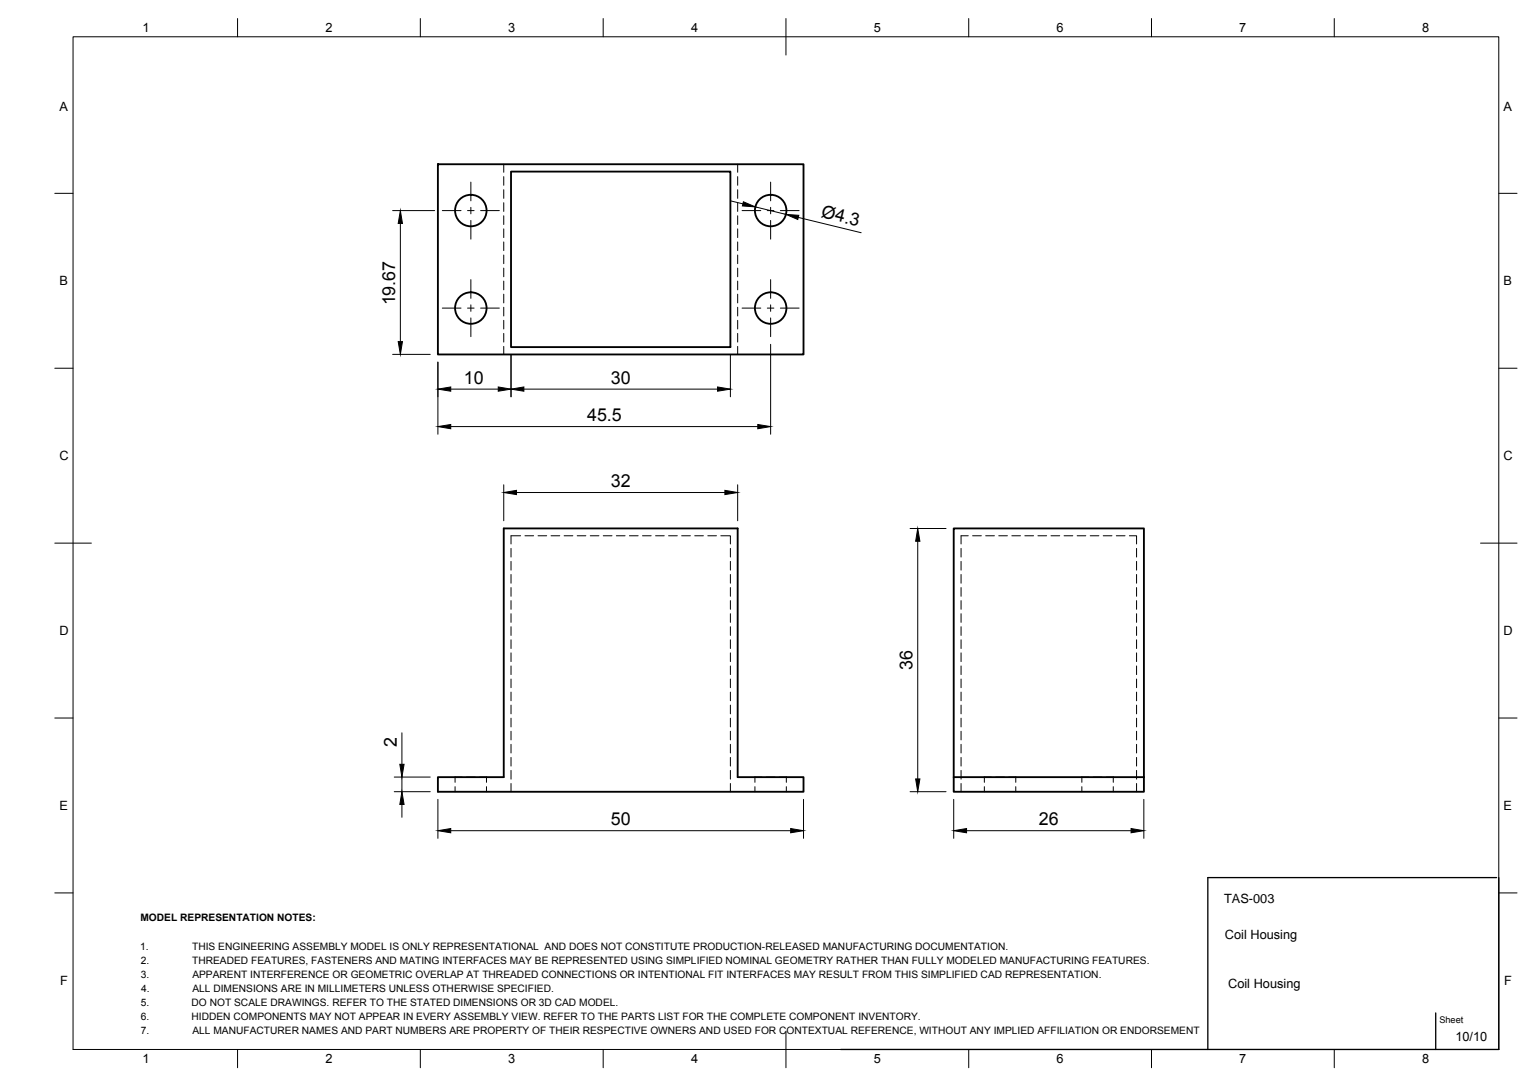
ISO-10303-21;
HEADER;
/* Generated by software containing ST-Developer
 * from STEP Tools, Inc. (www.steptools.com) 
 */

FILE_DESCRIPTION(
/* description */ ('STEP AP214'),
/* implementation_level */ '2;1');

FILE_NAME(
/* name */ 'Coil Housing.step',
/* time_stamp */ '2026-11-04T19:43:37-08:00',
/* author */ (''),
/* organization */ (''),
/* preprocessor_version */ 'ST-DEVELOPER v20.2',
/* originating_system */ 'Autodesk Translation Framework v15.17.0.0',
/* authorisation */ '');

FILE_SCHEMA (('AUTOMOTIVE_DESIGN { 1 0 10303 214 3 1 1 }'));
ENDSEC;

DATA;
#10=MECHANICAL_DESIGN_GEOMETRIC_PRESENTATION_REPRESENTATION('',(#134),#7627);
#86=TOROIDAL_SURFACE('',#2777,2.2,0.2);
#87=TOROIDAL_SURFACE('',#2781,2.2,0.2);
#88=TOROIDAL_SURFACE('',#2785,2.2,0.2);
#89=TOROIDAL_SURFACE('',#2789,2.2,0.2);
#104=SHAPE_REPRESENTATION_RELATIONSHIP('SRR','None',#7672,#113);
#113=ADVANCED_BREP_SHAPE_REPRESENTATION('',(#155),#7625);
#134=STYLED_ITEM('',(#7719),#155);
#155=MANIFOLD_SOLID_BREP('Body1',#2432);
#179=FACE_BOUND('',#605,.T.);
#180=FACE_BOUND('',#606,.T.);
#181=FACE_BOUND('',#607,.T.);
#182=FACE_BOUND('',#608,.T.);
#183=FACE_BOUND('',#609,.T.);
#184=FACE_BOUND('',#620,.T.);
#185=FACE_BOUND('',#621,.T.);
#186=FACE_BOUND('',#624,.T.);
#187=FACE_BOUND('',#625,.T.);
#222=PLANE('',#2801);
#223=PLANE('',#2802);
#224=PLANE('',#2803);
#225=PLANE('',#2804);
#226=PLANE('',#2805);
#227=PLANE('',#2806);
#228=PLANE('',#2807);
#229=PLANE('',#2808);
#230=PLANE('',#2809);
#231=PLANE('',#2810);
#232=PLANE('',#2811);
#233=PLANE('',#2812);
#234=PLANE('',#2813);
#235=PLANE('',#2814);
#236=PLANE('',#2815);
#302=CYLINDRICAL_SURFACE('',#2793,2.15);
#303=CYLINDRICAL_SURFACE('',#2795,2.15);
#304=CYLINDRICAL_SURFACE('',#2797,2.15);
#305=CYLINDRICAL_SURFACE('',#2799,2.15);
#418=FACE_OUTER_BOUND('',#594,.T.);
#419=FACE_OUTER_BOUND('',#595,.T.);
#420=FACE_OUTER_BOUND('',#596,.T.);
#421=FACE_OUTER_BOUND('',#597,.T.);
#422=FACE_OUTER_BOUND('',#598,.T.);
#423=FACE_OUTER_BOUND('',#599,.T.);
#424=FACE_OUTER_BOUND('',#600,.T.);
#425=FACE_OUTER_BOUND('',#601,.T.);
#426=FACE_OUTER_BOUND('',#602,.T.);
#427=FACE_OUTER_BOUND('',#603,.T.);
#428=FACE_OUTER_BOUND('',#604,.T.);
#429=FACE_OUTER_BOUND('',#610,.T.);
#430=FACE_OUTER_BOUND('',#611,.T.);
#431=FACE_OUTER_BOUND('',#612,.T.);
#432=FACE_OUTER_BOUND('',#613,.T.);
#433=FACE_OUTER_BOUND('',#614,.T.);
#434=FACE_OUTER_BOUND('',#615,.T.);
#435=FACE_OUTER_BOUND('',#616,.T.);
#436=FACE_OUTER_BOUND('',#617,.T.);
#437=FACE_OUTER_BOUND('',#618,.T.);
#438=FACE_OUTER_BOUND('',#619,.T.);
#439=FACE_OUTER_BOUND('',#622,.T.);
#440=FACE_OUTER_BOUND('',#623,.T.);
#594=EDGE_LOOP('',(#2057,#2058,#2059,#2060));
#595=EDGE_LOOP('',(#2061,#2062,#2063,#2064));
#596=EDGE_LOOP('',(#2065,#2066,#2067,#2068));
#597=EDGE_LOOP('',(#2069,#2070,#2071,#2072));
#598=EDGE_LOOP('',(#2073,#2074,#2075,#2076));
#599=EDGE_LOOP('',(#2077,#2078,#2079,#2080));
#600=EDGE_LOOP('',(#2081,#2082,#2083,#2084));
#601=EDGE_LOOP('',(#2085,#2086,#2087,#2088));
#602=EDGE_LOOP('',(#2089,#2090,#2091,#2092));
#603=EDGE_LOOP('',(#2093,#2094,#2095,#2096));
#604=EDGE_LOOP('',(#2097,#2098,#2099,#2100));
#605=EDGE_LOOP('',(#2101,#2102,#2103,#2104));
#606=EDGE_LOOP('',(#2105));
#607=EDGE_LOOP('',(#2106));
#608=EDGE_LOOP('',(#2107));
#609=EDGE_LOOP('',(#2108));
#610=EDGE_LOOP('',(#2109,#2110,#2111,#2112,#2113,#2114,#2115,#2116));
#611=EDGE_LOOP('',(#2117,#2118,#2119,#2120,#2121,#2122,#2123,#2124));
#612=EDGE_LOOP('',(#2125,#2126,#2127,#2128));
#613=EDGE_LOOP('',(#2129,#2130,#2131,#2132));
#614=EDGE_LOOP('',(#2133,#2134,#2135,#2136));
#615=EDGE_LOOP('',(#2137,#2138,#2139,#2140));
#616=EDGE_LOOP('',(#2141,#2142,#2143,#2144));
#617=EDGE_LOOP('',(#2145,#2146,#2147,#2148));
#618=EDGE_LOOP('',(#2149,#2150,#2151,#2152));
#619=EDGE_LOOP('',(#2153,#2154,#2155,#2156));
#620=EDGE_LOOP('',(#2157));
#621=EDGE_LOOP('',(#2158));
#622=EDGE_LOOP('',(#2159,#2160,#2161,#2162));
#623=EDGE_LOOP('',(#2163,#2164,#2165,#2166));
#624=EDGE_LOOP('',(#2167));
#625=EDGE_LOOP('',(#2168));
#773=CIRCLE('',#2778,2.15);
#774=CIRCLE('',#2779,0.2);
#775=CIRCLE('',#2780,2.2);
#776=CIRCLE('',#2782,2.15);
#777=CIRCLE('',#2783,0.2);
#778=CIRCLE('',#2784,2.2);
#779=CIRCLE('',#2786,2.15);
#780=CIRCLE('',#2787,0.2);
#781=CIRCLE('',#2788,2.2);
#782=CIRCLE('',#2790,2.15);
#783=CIRCLE('',#2791,0.2);
#784=CIRCLE('',#2792,2.2);
#785=CIRCLE('',#2794,2.15);
#786=CIRCLE('',#2796,2.15);
#787=CIRCLE('',#2798,2.15);
#788=CIRCLE('',#2800,2.15);
#891=LINE('',#7416,#1047);
#892=LINE('',#7420,#1048);
#893=LINE('',#7424,#1049);
#894=LINE('',#7428,#1050);
#895=LINE('',#7432,#1051);
#896=LINE('',#7434,#1052);
#897=LINE('',#7436,#1053);
#898=LINE('',#7437,#1054);
#899=LINE('',#7441,#1055);
#900=LINE('',#7443,#1056);
#901=LINE('',#7445,#1057);
#902=LINE('',#7446,#1058);
#903=LINE('',#7450,#1059);
#904=LINE('',#7452,#1060);
#905=LINE('',#7454,#1061);
#906=LINE('',#7455,#1062);
#907=LINE('',#7458,#1063);
#908=LINE('',#7460,#1064);
#909=LINE('',#7462,#1065);
#910=LINE('',#7463,#1066);
#911=LINE('',#7466,#1067);
#912=LINE('',#7467,#1068);
#913=LINE('',#7468,#1069);
#914=LINE('',#7470,#1070);
#915=LINE('',#7471,#1071);
#916=LINE('',#7474,#1072);
#917=LINE('',#7475,#1073);
#918=LINE('',#7476,#1074);
#919=LINE('',#7478,#1075);
#920=LINE('',#7479,#1076);
#921=LINE('',#7482,#1077);
#922=LINE('',#7484,#1078);
#923=LINE('',#7485,#1079);
#924=LINE('',#7488,#1080);
#925=LINE('',#7489,#1081);
#926=LINE('',#7492,#1082);
#927=LINE('',#7493,#1083);
#928=LINE('',#7495,#1084);
#929=LINE('',#7499,#1085);
#930=LINE('',#7502,#1086);
#1047=VECTOR('',#3474,2.15);
#1048=VECTOR('',#3479,2.15);
#1049=VECTOR('',#3484,2.15);
#1050=VECTOR('',#3489,2.15);
#1051=VECTOR('',#3492,1000.);
#1052=VECTOR('',#3493,1000.);
#1053=VECTOR('',#3494,1000.);
#1054=VECTOR('',#3495,1000.);
#1055=VECTOR('',#3498,1000.);
#1056=VECTOR('',#3499,1000.);
#1057=VECTOR('',#3500,1000.);
#1058=VECTOR('',#3501,1000.);
#1059=VECTOR('',#3504,1000.);
#1060=VECTOR('',#3505,1000.);
#1061=VECTOR('',#3506,1000.);
#1062=VECTOR('',#3507,1000.);
#1063=VECTOR('',#3508,1000.);
#1064=VECTOR('',#3509,1000.);
#1065=VECTOR('',#3510,1000.);
#1066=VECTOR('',#3511,1000.);
#1067=VECTOR('',#3514,1000.);
#1068=VECTOR('',#3515,1000.);
#1069=VECTOR('',#3516,1000.);
#1070=VECTOR('',#3517,1000.);
#1071=VECTOR('',#3518,1000.);
#1072=VECTOR('',#3521,1000.);
#1073=VECTOR('',#3522,1000.);
#1074=VECTOR('',#3523,1000.);
#1075=VECTOR('',#3524,1000.);
#1076=VECTOR('',#3525,1000.);
#1077=VECTOR('',#3528,1000.);
#1078=VECTOR('',#3529,1000.);
#1079=VECTOR('',#3530,1000.);
#1080=VECTOR('',#3533,1000.);
#1081=VECTOR('',#3534,1000.);
#1082=VECTOR('',#3537,1000.);
#1083=VECTOR('',#3538,1000.);
#1084=VECTOR('',#3541,1000.);
#1085=VECTOR('',#3548,1000.);
#1086=VECTOR('',#3553,1000.);
#1243=VERTEX_POINT('',#7390);
#1244=VERTEX_POINT('',#7392);
#1245=VERTEX_POINT('',#7396);
#1246=VERTEX_POINT('',#7398);
#1247=VERTEX_POINT('',#7402);
#1248=VERTEX_POINT('',#7404);
#1249=VERTEX_POINT('',#7408);
#1250=VERTEX_POINT('',#7410);
#1251=VERTEX_POINT('',#7414);
#1252=VERTEX_POINT('',#7418);
#1253=VERTEX_POINT('',#7422);
#1254=VERTEX_POINT('',#7426);
#1255=VERTEX_POINT('',#7430);
#1256=VERTEX_POINT('',#7431);
#1257=VERTEX_POINT('',#7433);
#1258=VERTEX_POINT('',#7435);
#1259=VERTEX_POINT('',#7439);
#1260=VERTEX_POINT('',#7440);
#1261=VERTEX_POINT('',#7442);
#1262=VERTEX_POINT('',#7444);
#1263=VERTEX_POINT('',#7448);
#1264=VERTEX_POINT('',#7449);
#1265=VERTEX_POINT('',#7451);
#1266=VERTEX_POINT('',#7453);
#1267=VERTEX_POINT('',#7456);
#1268=VERTEX_POINT('',#7457);
#1269=VERTEX_POINT('',#7459);
#1270=VERTEX_POINT('',#7461);
#1271=VERTEX_POINT('',#7465);
#1272=VERTEX_POINT('',#7469);
#1273=VERTEX_POINT('',#7473);
#1274=VERTEX_POINT('',#7477);
#1275=VERTEX_POINT('',#7481);
#1276=VERTEX_POINT('',#7483);
#1277=VERTEX_POINT('',#7487);
#1278=VERTEX_POINT('',#7491);
#1523=EDGE_CURVE('',#1243,#1243,#773,.T.);
#1524=EDGE_CURVE('',#1243,#1244,#774,.T.);
#1525=EDGE_CURVE('',#1244,#1244,#775,.T.);
#1526=EDGE_CURVE('',#1245,#1245,#776,.T.);
#1527=EDGE_CURVE('',#1245,#1246,#777,.T.);
#1528=EDGE_CURVE('',#1246,#1246,#778,.T.);
#1529=EDGE_CURVE('',#1247,#1247,#779,.T.);
#1530=EDGE_CURVE('',#1247,#1248,#780,.T.);
#1531=EDGE_CURVE('',#1248,#1248,#781,.T.);
#1532=EDGE_CURVE('',#1249,#1249,#782,.T.);
#1533=EDGE_CURVE('',#1249,#1250,#783,.T.);
#1534=EDGE_CURVE('',#1250,#1250,#784,.T.);
#1535=EDGE_CURVE('',#1251,#1251,#785,.T.);
#1536=EDGE_CURVE('',#1251,#1249,#891,.T.);
#1537=EDGE_CURVE('',#1252,#1252,#786,.T.);
#1538=EDGE_CURVE('',#1252,#1247,#892,.T.);
#1539=EDGE_CURVE('',#1253,#1253,#787,.T.);
#1540=EDGE_CURVE('',#1253,#1245,#893,.T.);
#1541=EDGE_CURVE('',#1254,#1254,#788,.T.);
#1542=EDGE_CURVE('',#1254,#1243,#894,.T.);
#1543=EDGE_CURVE('',#1255,#1256,#895,.T.);
#1544=EDGE_CURVE('',#1257,#1255,#896,.T.);
#1545=EDGE_CURVE('',#1258,#1257,#897,.T.);
#1546=EDGE_CURVE('',#1258,#1256,#898,.T.);
#1547=EDGE_CURVE('',#1259,#1260,#899,.T.);
#1548=EDGE_CURVE('',#1261,#1259,#900,.T.);
#1549=EDGE_CURVE('',#1262,#1261,#901,.T.);
#1550=EDGE_CURVE('',#1262,#1260,#902,.T.);
#1551=EDGE_CURVE('',#1263,#1264,#903,.T.);
#1552=EDGE_CURVE('',#1265,#1263,#904,.T.);
#1553=EDGE_CURVE('',#1266,#1265,#905,.T.);
#1554=EDGE_CURVE('',#1264,#1266,#906,.T.);
#1555=EDGE_CURVE('',#1267,#1268,#907,.T.);
#1556=EDGE_CURVE('',#1268,#1269,#908,.T.);
#1557=EDGE_CURVE('',#1269,#1270,#909,.T.);
#1558=EDGE_CURVE('',#1270,#1267,#910,.T.);
#1559=EDGE_CURVE('',#1271,#1264,#911,.T.);
#1560=EDGE_CURVE('',#1256,#1271,#912,.T.);
#1561=EDGE_CURVE('',#1261,#1258,#913,.T.);
#1562=EDGE_CURVE('',#1272,#1259,#914,.T.);
#1563=EDGE_CURVE('',#1272,#1263,#915,.T.);
#1564=EDGE_CURVE('',#1273,#1265,#916,.T.);
#1565=EDGE_CURVE('',#1260,#1273,#917,.T.);
#1566=EDGE_CURVE('',#1257,#1262,#918,.T.);
#1567=EDGE_CURVE('',#1274,#1255,#919,.T.);
#1568=EDGE_CURVE('',#1274,#1266,#920,.T.);
#1569=EDGE_CURVE('',#1275,#1267,#921,.T.);
#1570=EDGE_CURVE('',#1275,#1276,#922,.T.);
#1571=EDGE_CURVE('',#1276,#1268,#923,.T.);
#1572=EDGE_CURVE('',#1276,#1277,#924,.T.);
#1573=EDGE_CURVE('',#1277,#1269,#925,.T.);
#1574=EDGE_CURVE('',#1277,#1278,#926,.T.);
#1575=EDGE_CURVE('',#1278,#1270,#927,.T.);
#1576=EDGE_CURVE('',#1278,#1275,#928,.T.);
#1577=EDGE_CURVE('',#1273,#1272,#929,.T.);
#1578=EDGE_CURVE('',#1271,#1274,#930,.T.);
#2057=ORIENTED_EDGE('',*,*,#1523,.T.);
#2058=ORIENTED_EDGE('',*,*,#1524,.T.);
#2059=ORIENTED_EDGE('',*,*,#1525,.T.);
#2060=ORIENTED_EDGE('',*,*,#1524,.F.);
#2061=ORIENTED_EDGE('',*,*,#1526,.T.);
#2062=ORIENTED_EDGE('',*,*,#1527,.T.);
#2063=ORIENTED_EDGE('',*,*,#1528,.T.);
#2064=ORIENTED_EDGE('',*,*,#1527,.F.);
#2065=ORIENTED_EDGE('',*,*,#1529,.T.);
#2066=ORIENTED_EDGE('',*,*,#1530,.T.);
#2067=ORIENTED_EDGE('',*,*,#1531,.T.);
#2068=ORIENTED_EDGE('',*,*,#1530,.F.);
#2069=ORIENTED_EDGE('',*,*,#1532,.T.);
#2070=ORIENTED_EDGE('',*,*,#1533,.T.);
#2071=ORIENTED_EDGE('',*,*,#1534,.T.);
#2072=ORIENTED_EDGE('',*,*,#1533,.F.);
#2073=ORIENTED_EDGE('',*,*,#1535,.F.);
#2074=ORIENTED_EDGE('',*,*,#1536,.T.);
#2075=ORIENTED_EDGE('',*,*,#1532,.F.);
#2076=ORIENTED_EDGE('',*,*,#1536,.F.);
#2077=ORIENTED_EDGE('',*,*,#1537,.F.);
#2078=ORIENTED_EDGE('',*,*,#1538,.T.);
#2079=ORIENTED_EDGE('',*,*,#1529,.F.);
#2080=ORIENTED_EDGE('',*,*,#1538,.F.);
#2081=ORIENTED_EDGE('',*,*,#1539,.F.);
#2082=ORIENTED_EDGE('',*,*,#1540,.T.);
#2083=ORIENTED_EDGE('',*,*,#1526,.F.);
#2084=ORIENTED_EDGE('',*,*,#1540,.F.);
#2085=ORIENTED_EDGE('',*,*,#1541,.F.);
#2086=ORIENTED_EDGE('',*,*,#1542,.T.);
#2087=ORIENTED_EDGE('',*,*,#1523,.F.);
#2088=ORIENTED_EDGE('',*,*,#1542,.F.);
#2089=ORIENTED_EDGE('',*,*,#1543,.F.);
#2090=ORIENTED_EDGE('',*,*,#1544,.F.);
#2091=ORIENTED_EDGE('',*,*,#1545,.F.);
#2092=ORIENTED_EDGE('',*,*,#1546,.T.);
#2093=ORIENTED_EDGE('',*,*,#1547,.F.);
#2094=ORIENTED_EDGE('',*,*,#1548,.F.);
#2095=ORIENTED_EDGE('',*,*,#1549,.F.);
#2096=ORIENTED_EDGE('',*,*,#1550,.T.);
#2097=ORIENTED_EDGE('',*,*,#1551,.F.);
#2098=ORIENTED_EDGE('',*,*,#1552,.F.);
#2099=ORIENTED_EDGE('',*,*,#1553,.F.);
#2100=ORIENTED_EDGE('',*,*,#1554,.F.);
#2101=ORIENTED_EDGE('',*,*,#1555,.T.);
#2102=ORIENTED_EDGE('',*,*,#1556,.T.);
#2103=ORIENTED_EDGE('',*,*,#1557,.T.);
#2104=ORIENTED_EDGE('',*,*,#1558,.T.);
#2105=ORIENTED_EDGE('',*,*,#1535,.T.);
#2106=ORIENTED_EDGE('',*,*,#1537,.T.);
#2107=ORIENTED_EDGE('',*,*,#1539,.T.);
#2108=ORIENTED_EDGE('',*,*,#1541,.T.);
#2109=ORIENTED_EDGE('',*,*,#1551,.T.);
#2110=ORIENTED_EDGE('',*,*,#1559,.F.);
#2111=ORIENTED_EDGE('',*,*,#1560,.F.);
#2112=ORIENTED_EDGE('',*,*,#1546,.F.);
#2113=ORIENTED_EDGE('',*,*,#1561,.F.);
#2114=ORIENTED_EDGE('',*,*,#1548,.T.);
#2115=ORIENTED_EDGE('',*,*,#1562,.F.);
#2116=ORIENTED_EDGE('',*,*,#1563,.T.);
#2117=ORIENTED_EDGE('',*,*,#1553,.T.);
#2118=ORIENTED_EDGE('',*,*,#1564,.F.);
#2119=ORIENTED_EDGE('',*,*,#1565,.F.);
#2120=ORIENTED_EDGE('',*,*,#1550,.F.);
#2121=ORIENTED_EDGE('',*,*,#1566,.F.);
#2122=ORIENTED_EDGE('',*,*,#1544,.T.);
#2123=ORIENTED_EDGE('',*,*,#1567,.F.);
#2124=ORIENTED_EDGE('',*,*,#1568,.T.);
#2125=ORIENTED_EDGE('',*,*,#1555,.F.);
#2126=ORIENTED_EDGE('',*,*,#1569,.F.);
#2127=ORIENTED_EDGE('',*,*,#1570,.T.);
#2128=ORIENTED_EDGE('',*,*,#1571,.T.);
#2129=ORIENTED_EDGE('',*,*,#1556,.F.);
#2130=ORIENTED_EDGE('',*,*,#1571,.F.);
#2131=ORIENTED_EDGE('',*,*,#1572,.T.);
#2132=ORIENTED_EDGE('',*,*,#1573,.T.);
#2133=ORIENTED_EDGE('',*,*,#1557,.F.);
#2134=ORIENTED_EDGE('',*,*,#1573,.F.);
#2135=ORIENTED_EDGE('',*,*,#1574,.T.);
#2136=ORIENTED_EDGE('',*,*,#1575,.T.);
#2137=ORIENTED_EDGE('',*,*,#1558,.F.);
#2138=ORIENTED_EDGE('',*,*,#1575,.F.);
#2139=ORIENTED_EDGE('',*,*,#1576,.T.);
#2140=ORIENTED_EDGE('',*,*,#1569,.T.);
#2141=ORIENTED_EDGE('',*,*,#1572,.F.);
#2142=ORIENTED_EDGE('',*,*,#1570,.F.);
#2143=ORIENTED_EDGE('',*,*,#1576,.F.);
#2144=ORIENTED_EDGE('',*,*,#1574,.F.);
#2145=ORIENTED_EDGE('',*,*,#1561,.T.);
#2146=ORIENTED_EDGE('',*,*,#1545,.T.);
#2147=ORIENTED_EDGE('',*,*,#1566,.T.);
#2148=ORIENTED_EDGE('',*,*,#1549,.T.);
#2149=ORIENTED_EDGE('',*,*,#1552,.T.);
#2150=ORIENTED_EDGE('',*,*,#1563,.F.);
#2151=ORIENTED_EDGE('',*,*,#1577,.F.);
#2152=ORIENTED_EDGE('',*,*,#1564,.T.);
#2153=ORIENTED_EDGE('',*,*,#1547,.T.);
#2154=ORIENTED_EDGE('',*,*,#1565,.T.);
#2155=ORIENTED_EDGE('',*,*,#1577,.T.);
#2156=ORIENTED_EDGE('',*,*,#1562,.T.);
#2157=ORIENTED_EDGE('',*,*,#1531,.F.);
#2158=ORIENTED_EDGE('',*,*,#1534,.F.);
#2159=ORIENTED_EDGE('',*,*,#1554,.T.);
#2160=ORIENTED_EDGE('',*,*,#1568,.F.);
#2161=ORIENTED_EDGE('',*,*,#1578,.F.);
#2162=ORIENTED_EDGE('',*,*,#1559,.T.);
#2163=ORIENTED_EDGE('',*,*,#1567,.T.);
#2164=ORIENTED_EDGE('',*,*,#1543,.T.);
#2165=ORIENTED_EDGE('',*,*,#1560,.T.);
#2166=ORIENTED_EDGE('',*,*,#1578,.T.);
#2167=ORIENTED_EDGE('',*,*,#1525,.F.);
#2168=ORIENTED_EDGE('',*,*,#1528,.F.);
#2369=ADVANCED_FACE('',(#418),#86,.T.);
#2370=ADVANCED_FACE('',(#419),#87,.T.);
#2371=ADVANCED_FACE('',(#420),#88,.T.);
#2372=ADVANCED_FACE('',(#421),#89,.T.);
#2373=ADVANCED_FACE('',(#422),#302,.F.);
#2374=ADVANCED_FACE('',(#423),#303,.F.);
#2375=ADVANCED_FACE('',(#424),#304,.F.);
#2376=ADVANCED_FACE('',(#425),#305,.F.);
#2377=ADVANCED_FACE('',(#426),#222,.F.);
#2378=ADVANCED_FACE('',(#427),#223,.F.);
#2379=ADVANCED_FACE('',(#428,#179,#180,#181,#182,#183),#224,.F.);
#2380=ADVANCED_FACE('',(#429),#225,.F.);
#2381=ADVANCED_FACE('',(#430),#226,.F.);
#2382=ADVANCED_FACE('',(#431),#227,.T.);
#2383=ADVANCED_FACE('',(#432),#228,.T.);
#2384=ADVANCED_FACE('',(#433),#229,.T.);
#2385=ADVANCED_FACE('',(#434),#230,.T.);
#2386=ADVANCED_FACE('',(#435),#231,.T.);
#2387=ADVANCED_FACE('',(#436),#232,.F.);
#2388=ADVANCED_FACE('',(#437),#233,.F.);
#2389=ADVANCED_FACE('',(#438,#184,#185),#234,.F.);
#2390=ADVANCED_FACE('',(#439),#235,.F.);
#2391=ADVANCED_FACE('',(#440,#186,#187),#236,.F.);
#2432=CLOSED_SHELL('',(#2369,#2370,#2371,#2372,#2373,#2374,#2375,#2376,
#2377,#2378,#2379,#2380,#2381,#2382,#2383,#2384,#2385,#2386,#2387,#2388,
#2389,#2390,#2391));
#2776=AXIS2_PLACEMENT_3D('',#7388,#3436,#3437);
#2777=AXIS2_PLACEMENT_3D('',#7389,#3438,#3439);
#2778=AXIS2_PLACEMENT_3D('',#7391,#3440,#3441);
#2779=AXIS2_PLACEMENT_3D('',#7393,#3442,#3443);
#2780=AXIS2_PLACEMENT_3D('',#7394,#3444,#3445);
#2781=AXIS2_PLACEMENT_3D('',#7395,#3446,#3447);
#2782=AXIS2_PLACEMENT_3D('',#7397,#3448,#3449);
#2783=AXIS2_PLACEMENT_3D('',#7399,#3450,#3451);
#2784=AXIS2_PLACEMENT_3D('',#7400,#3452,#3453);
#2785=AXIS2_PLACEMENT_3D('',#7401,#3454,#3455);
#2786=AXIS2_PLACEMENT_3D('',#7403,#3456,#3457);
#2787=AXIS2_PLACEMENT_3D('',#7405,#3458,#3459);
#2788=AXIS2_PLACEMENT_3D('',#7406,#3460,#3461);
#2789=AXIS2_PLACEMENT_3D('',#7407,#3462,#3463);
#2790=AXIS2_PLACEMENT_3D('',#7409,#3464,#3465);
#2791=AXIS2_PLACEMENT_3D('',#7411,#3466,#3467);
#2792=AXIS2_PLACEMENT_3D('',#7412,#3468,#3469);
#2793=AXIS2_PLACEMENT_3D('',#7413,#3470,#3471);
#2794=AXIS2_PLACEMENT_3D('',#7415,#3472,#3473);
#2795=AXIS2_PLACEMENT_3D('',#7417,#3475,#3476);
#2796=AXIS2_PLACEMENT_3D('',#7419,#3477,#3478);
#2797=AXIS2_PLACEMENT_3D('',#7421,#3480,#3481);
#2798=AXIS2_PLACEMENT_3D('',#7423,#3482,#3483);
#2799=AXIS2_PLACEMENT_3D('',#7425,#3485,#3486);
#2800=AXIS2_PLACEMENT_3D('',#7427,#3487,#3488);
#2801=AXIS2_PLACEMENT_3D('',#7429,#3490,#3491);
#2802=AXIS2_PLACEMENT_3D('',#7438,#3496,#3497);
#2803=AXIS2_PLACEMENT_3D('',#7447,#3502,#3503);
#2804=AXIS2_PLACEMENT_3D('',#7464,#3512,#3513);
#2805=AXIS2_PLACEMENT_3D('',#7472,#3519,#3520);
#2806=AXIS2_PLACEMENT_3D('',#7480,#3526,#3527);
#2807=AXIS2_PLACEMENT_3D('',#7486,#3531,#3532);
#2808=AXIS2_PLACEMENT_3D('',#7490,#3535,#3536);
#2809=AXIS2_PLACEMENT_3D('',#7494,#3539,#3540);
#2810=AXIS2_PLACEMENT_3D('',#7496,#3542,#3543);
#2811=AXIS2_PLACEMENT_3D('',#7497,#3544,#3545);
#2812=AXIS2_PLACEMENT_3D('',#7498,#3546,#3547);
#2813=AXIS2_PLACEMENT_3D('',#7500,#3549,#3550);
#2814=AXIS2_PLACEMENT_3D('',#7501,#3551,#3552);
#2815=AXIS2_PLACEMENT_3D('',#7503,#3554,#3555);
#3436=DIRECTION('axis',(0.,0.,1.));
#3437=DIRECTION('refdir',(1.,0.,0.));
#3438=DIRECTION('center_axis',(0.,1.,0.));
#3439=DIRECTION('ref_axis',(0.,0.,1.));
#3440=DIRECTION('center_axis',(0.,-1.,0.));
#3441=DIRECTION('ref_axis',(0.,0.,-1.));
#3442=DIRECTION('center_axis',(-1.,0.,0.));
#3443=DIRECTION('ref_axis',(0.,0.,-1.));
#3444=DIRECTION('center_axis',(0.,1.,0.));
#3445=DIRECTION('ref_axis',(0.,0.,1.));
#3446=DIRECTION('center_axis',(0.,1.,0.));
#3447=DIRECTION('ref_axis',(0.,0.,1.));
#3448=DIRECTION('center_axis',(0.,-1.,0.));
#3449=DIRECTION('ref_axis',(0.,0.,-1.));
#3450=DIRECTION('center_axis',(-1.,0.,0.));
#3451=DIRECTION('ref_axis',(0.,0.,-1.));
#3452=DIRECTION('center_axis',(0.,1.,0.));
#3453=DIRECTION('ref_axis',(0.,0.,1.));
#3454=DIRECTION('center_axis',(0.,1.,0.));
#3455=DIRECTION('ref_axis',(0.,0.,1.));
#3456=DIRECTION('center_axis',(0.,-1.,0.));
#3457=DIRECTION('ref_axis',(0.,0.,-1.));
#3458=DIRECTION('center_axis',(-1.,0.,0.));
#3459=DIRECTION('ref_axis',(0.,0.,-1.));
#3460=DIRECTION('center_axis',(0.,1.,0.));
#3461=DIRECTION('ref_axis',(0.,0.,1.));
#3462=DIRECTION('center_axis',(0.,1.,0.));
#3463=DIRECTION('ref_axis',(0.,0.,1.));
#3464=DIRECTION('center_axis',(0.,-1.,0.));
#3465=DIRECTION('ref_axis',(0.,0.,-1.));
#3466=DIRECTION('center_axis',(-1.,0.,0.));
#3467=DIRECTION('ref_axis',(0.,0.,-1.));
#3468=DIRECTION('center_axis',(0.,1.,0.));
#3469=DIRECTION('ref_axis',(0.,0.,1.));
#3470=DIRECTION('center_axis',(0.,1.,0.));
#3471=DIRECTION('ref_axis',(0.,0.,1.));
#3472=DIRECTION('center_axis',(0.,1.,0.));
#3473=DIRECTION('ref_axis',(0.,0.,1.));
#3474=DIRECTION('',(0.,1.,0.));
#3475=DIRECTION('center_axis',(0.,1.,0.));
#3476=DIRECTION('ref_axis',(0.,0.,1.));
#3477=DIRECTION('center_axis',(0.,1.,0.));
#3478=DIRECTION('ref_axis',(0.,0.,1.));
#3479=DIRECTION('',(0.,1.,0.));
#3480=DIRECTION('center_axis',(0.,1.,0.));
#3481=DIRECTION('ref_axis',(0.,0.,1.));
#3482=DIRECTION('center_axis',(0.,1.,0.));
#3483=DIRECTION('ref_axis',(0.,0.,1.));
#3484=DIRECTION('',(0.,1.,0.));
#3485=DIRECTION('center_axis',(0.,1.,0.));
#3486=DIRECTION('ref_axis',(0.,0.,1.));
#3487=DIRECTION('center_axis',(0.,1.,0.));
#3488=DIRECTION('ref_axis',(0.,0.,1.));
#3489=DIRECTION('',(0.,1.,0.));
#3490=DIRECTION('center_axis',(0.,0.,1.));
#3491=DIRECTION('ref_axis',(1.,0.,0.));
#3492=DIRECTION('',(1.,0.,0.));
#3493=DIRECTION('',(0.,-1.,0.));
#3494=DIRECTION('',(-1.,0.,0.));
#3495=DIRECTION('',(0.,-1.,0.));
#3496=DIRECTION('center_axis',(0.,0.,-1.));
#3497=DIRECTION('ref_axis',(-1.,0.,0.));
#3498=DIRECTION('',(-1.,0.,0.));
#3499=DIRECTION('',(0.,-1.,0.));
#3500=DIRECTION('',(1.,0.,0.));
#3501=DIRECTION('',(0.,-1.,0.));
#3502=DIRECTION('center_axis',(0.,1.,0.));
#3503=DIRECTION('ref_axis',(0.,0.,1.));
#3504=DIRECTION('',(0.,0.,-1.));
#3505=DIRECTION('',(1.,0.,0.));
#3506=DIRECTION('',(0.,0.,1.));
#3507=DIRECTION('',(-1.,0.,0.));
#3508=DIRECTION('',(0.,0.,-1.));
#3509=DIRECTION('',(-1.,0.,0.));
#3510=DIRECTION('',(0.,0.,1.));
#3511=DIRECTION('',(1.,0.,0.));
#3512=DIRECTION('center_axis',(-1.,0.,0.));
#3513=DIRECTION('ref_axis',(0.,0.,1.));
#3514=DIRECTION('',(0.,-1.,0.));
#3515=DIRECTION('',(0.,0.,-1.));
#3516=DIRECTION('',(0.,0.,-1.));
#3517=DIRECTION('',(0.,0.,-1.));
#3518=DIRECTION('',(0.,-1.,0.));
#3519=DIRECTION('center_axis',(1.,0.,0.));
#3520=DIRECTION('ref_axis',(0.,0.,-1.));
#3521=DIRECTION('',(0.,-1.,0.));
#3522=DIRECTION('',(0.,0.,1.));
#3523=DIRECTION('',(0.,0.,1.));
#3524=DIRECTION('',(0.,0.,1.));
#3525=DIRECTION('',(0.,-1.,0.));
#3526=DIRECTION('center_axis',(-1.,0.,0.));
#3527=DIRECTION('ref_axis',(0.,0.,1.));
#3528=DIRECTION('',(0.,-1.,0.));
#3529=DIRECTION('',(0.,0.,-1.));
#3530=DIRECTION('',(0.,-1.,0.));
#3531=DIRECTION('center_axis',(0.,0.,1.));
#3532=DIRECTION('ref_axis',(1.,0.,0.));
#3533=DIRECTION('',(-1.,0.,0.));
#3534=DIRECTION('',(0.,-1.,0.));
#3535=DIRECTION('center_axis',(1.,0.,0.));
#3536=DIRECTION('ref_axis',(0.,0.,-1.));
#3537=DIRECTION('',(0.,0.,1.));
#3538=DIRECTION('',(0.,-1.,0.));
#3539=DIRECTION('center_axis',(0.,0.,-1.));
#3540=DIRECTION('ref_axis',(-1.,0.,0.));
#3541=DIRECTION('',(1.,0.,0.));
#3542=DIRECTION('center_axis',(0.,-1.,0.));
#3543=DIRECTION('ref_axis',(0.,0.,-1.));
#3544=DIRECTION('center_axis',(0.,-1.,0.));
#3545=DIRECTION('ref_axis',(0.,0.,-1.));
#3546=DIRECTION('center_axis',(0.,0.,-1.));
#3547=DIRECTION('ref_axis',(-1.,0.,0.));
#3548=DIRECTION('',(1.,0.,0.));
#3549=DIRECTION('center_axis',(0.,-1.,0.));
#3550=DIRECTION('ref_axis',(0.,0.,-1.));
#3551=DIRECTION('center_axis',(0.,0.,1.));
#3552=DIRECTION('ref_axis',(1.,0.,0.));
#3553=DIRECTION('',(-1.,0.,0.));
#3554=DIRECTION('center_axis',(0.,-1.,0.));
#3555=DIRECTION('ref_axis',(0.,0.,-1.));
#7388=CARTESIAN_POINT('',(0.,0.,0.));
#7389=CARTESIAN_POINT('Origin',(-6.66666666666667,14.8,-20.5));
#7390=CARTESIAN_POINT('',(-6.66666666666667,14.9936491673104,-22.65));
#7391=CARTESIAN_POINT('Origin',(-6.66666666666667,14.9936491673104,-20.5));
#7392=CARTESIAN_POINT('',(-6.66666666666667,15.,-22.7));
#7393=CARTESIAN_POINT('Origin',(-6.66666666666667,14.8,-22.7));
#7394=CARTESIAN_POINT('Origin',(-6.66666666666667,15.,-20.5));
#7395=CARTESIAN_POINT('Origin',(6.66666666666666,14.8,-20.5));
#7396=CARTESIAN_POINT('',(6.66666666666666,14.9936491673104,-22.65));
#7397=CARTESIAN_POINT('Origin',(6.66666666666666,14.9936491673104,-20.5));
#7398=CARTESIAN_POINT('',(6.66666666666666,15.,-22.7));
#7399=CARTESIAN_POINT('Origin',(6.66666666666666,14.8,-22.7));
#7400=CARTESIAN_POINT('Origin',(6.66666666666666,15.,-20.5));
#7401=CARTESIAN_POINT('Origin',(6.66666666666666,14.8,20.5));
#7402=CARTESIAN_POINT('',(6.66666666666666,14.9936491673104,18.35));
#7403=CARTESIAN_POINT('Origin',(6.66666666666666,14.9936491673104,20.5));
#7404=CARTESIAN_POINT('',(6.66666666666666,15.,18.3));
#7405=CARTESIAN_POINT('Origin',(6.66666666666666,14.8,18.3));
#7406=CARTESIAN_POINT('Origin',(6.66666666666666,15.,20.5));
#7407=CARTESIAN_POINT('Origin',(-6.66666666666667,14.8,20.5));
#7408=CARTESIAN_POINT('',(-6.66666666666667,14.9936491673104,18.35));
#7409=CARTESIAN_POINT('Origin',(-6.66666666666667,14.9936491673104,20.5));
#7410=CARTESIAN_POINT('',(-6.66666666666667,15.,18.3));
#7411=CARTESIAN_POINT('Origin',(-6.66666666666667,14.8,18.3));
#7412=CARTESIAN_POINT('Origin',(-6.66666666666667,15.,20.5));
#7413=CARTESIAN_POINT('Origin',(-6.66666666666667,15.,20.5));
#7414=CARTESIAN_POINT('',(-6.66666666666667,13.,18.35));
#7415=CARTESIAN_POINT('Origin',(-6.66666666666667,13.,20.5));
#7416=CARTESIAN_POINT('',(-6.66666666666667,15.,18.35));
#7417=CARTESIAN_POINT('Origin',(6.66666666666666,15.,20.5));
#7418=CARTESIAN_POINT('',(6.66666666666666,13.,18.35));
#7419=CARTESIAN_POINT('Origin',(6.66666666666666,13.,20.5));
#7420=CARTESIAN_POINT('',(6.66666666666666,15.,18.35));
#7421=CARTESIAN_POINT('Origin',(6.66666666666666,15.,-20.5));
#7422=CARTESIAN_POINT('',(6.66666666666666,13.,-22.65));
#7423=CARTESIAN_POINT('Origin',(6.66666666666666,13.,-20.5));
#7424=CARTESIAN_POINT('',(6.66666666666666,15.,-22.65));
#7425=CARTESIAN_POINT('Origin',(-6.66666666666667,15.,-20.5));
#7426=CARTESIAN_POINT('',(-6.66666666666667,13.,-22.65));
#7427=CARTESIAN_POINT('Origin',(-6.66666666666667,13.,-20.5));
#7428=CARTESIAN_POINT('',(-6.66666666666667,15.,-22.65));
#7429=CARTESIAN_POINT('Origin',(0.,48.,-16.));
#7430=CARTESIAN_POINT('',(-13.,15.,-16.));
#7431=CARTESIAN_POINT('',(13.,15.,-16.));
#7432=CARTESIAN_POINT('',(-13.,15.,-16.));
#7433=CARTESIAN_POINT('',(-13.,49.,-16.));
#7434=CARTESIAN_POINT('',(-13.,48.,-16.));
#7435=CARTESIAN_POINT('',(13.,49.,-16.));
#7436=CARTESIAN_POINT('',(-13.,49.,-16.));
#7437=CARTESIAN_POINT('',(13.,48.,-16.));
#7438=CARTESIAN_POINT('Origin',(0.,48.,16.));
#7439=CARTESIAN_POINT('',(13.,15.,16.));
#7440=CARTESIAN_POINT('',(-13.,15.,16.));
#7441=CARTESIAN_POINT('',(-13.,15.,16.));
#7442=CARTESIAN_POINT('',(13.,49.,16.));
#7443=CARTESIAN_POINT('',(13.,48.,16.));
#7444=CARTESIAN_POINT('',(-13.,49.,16.));
#7445=CARTESIAN_POINT('',(-13.,49.,16.));
#7446=CARTESIAN_POINT('',(-13.,48.,16.));
#7447=CARTESIAN_POINT('Origin',(0.,13.,0.));
#7448=CARTESIAN_POINT('',(13.,13.,25.));
#7449=CARTESIAN_POINT('',(13.,13.,-25.));
#7450=CARTESIAN_POINT('',(13.,13.,0.));
#7451=CARTESIAN_POINT('',(-13.,13.,25.));
#7452=CARTESIAN_POINT('',(-13.,13.,25.));
#7453=CARTESIAN_POINT('',(-13.,13.,-25.));
#7454=CARTESIAN_POINT('',(-13.,13.,0.));
#7455=CARTESIAN_POINT('',(-13.,13.,-25.));
#7456=CARTESIAN_POINT('',(12.,13.,15.));
#7457=CARTESIAN_POINT('',(12.,13.,-15.));
#7458=CARTESIAN_POINT('',(12.,13.,15.));
#7459=CARTESIAN_POINT('',(-12.,13.,-15.));
#7460=CARTESIAN_POINT('',(-12.,13.,-15.));
#7461=CARTESIAN_POINT('',(-12.,13.,15.));
#7462=CARTESIAN_POINT('',(-12.,13.,15.));
#7463=CARTESIAN_POINT('',(-12.,13.,15.));
#7464=CARTESIAN_POINT('Origin',(13.,48.,0.));
#7465=CARTESIAN_POINT('',(13.,15.,-25.));
#7466=CARTESIAN_POINT('',(13.,15.,-25.));
#7467=CARTESIAN_POINT('',(13.,15.,-16.));
#7468=CARTESIAN_POINT('',(13.,49.,16.));
#7469=CARTESIAN_POINT('',(13.,15.,25.));
#7470=CARTESIAN_POINT('',(13.,15.,16.));
#7471=CARTESIAN_POINT('',(13.,15.,25.));
#7472=CARTESIAN_POINT('Origin',(-13.,48.,0.));
#7473=CARTESIAN_POINT('',(-13.,15.,25.));
#7474=CARTESIAN_POINT('',(-13.,15.,25.));
#7475=CARTESIAN_POINT('',(-13.,15.,16.));
#7476=CARTESIAN_POINT('',(-13.,49.,16.));
#7477=CARTESIAN_POINT('',(-13.,15.,-25.));
#7478=CARTESIAN_POINT('',(-13.,15.,-16.));
#7479=CARTESIAN_POINT('',(-13.,15.,-25.));
#7480=CARTESIAN_POINT('Origin',(12.,48.,15.));
#7481=CARTESIAN_POINT('',(12.,48.,15.));
#7482=CARTESIAN_POINT('',(12.,48.,15.));
#7483=CARTESIAN_POINT('',(12.,48.,-15.));
#7484=CARTESIAN_POINT('',(12.,48.,15.));
#7485=CARTESIAN_POINT('',(12.,48.,-15.));
#7486=CARTESIAN_POINT('Origin',(-12.,48.,-15.));
#7487=CARTESIAN_POINT('',(-12.,48.,-15.));
#7488=CARTESIAN_POINT('',(-12.,48.,-15.));
#7489=CARTESIAN_POINT('',(-12.,48.,-15.));
#7490=CARTESIAN_POINT('Origin',(-12.,48.,15.));
#7491=CARTESIAN_POINT('',(-12.,48.,15.));
#7492=CARTESIAN_POINT('',(-12.,48.,15.));
#7493=CARTESIAN_POINT('',(-12.,48.,15.));
#7494=CARTESIAN_POINT('Origin',(-12.,48.,15.));
#7495=CARTESIAN_POINT('',(-12.,48.,15.));
#7496=CARTESIAN_POINT('Origin',(0.,48.,0.));
#7497=CARTESIAN_POINT('Origin',(0.,49.,0.));
#7498=CARTESIAN_POINT('Origin',(-13.,15.,25.));
#7499=CARTESIAN_POINT('',(-13.,15.,25.));
#7500=CARTESIAN_POINT('Origin',(0.,15.,0.));
#7501=CARTESIAN_POINT('Origin',(-13.,15.,-25.));
#7502=CARTESIAN_POINT('',(-13.,15.,-25.));
#7503=CARTESIAN_POINT('Origin',(0.,15.,0.));
#7614=UNCERTAINTY_MEASURE_WITH_UNIT(LENGTH_MEASURE(0.01),#7628,
'DISTANCE_ACCURACY_VALUE',
'Maximum model space distance between geometric entities at asserted c
onnectivities');
#7616=UNCERTAINTY_MEASURE_WITH_UNIT(LENGTH_MEASURE(0.01),#7628,
'DISTANCE_ACCURACY_VALUE',
'Maximum model space distance between geometric entities at asserted c
onnectivities');
#7625=(
GEOMETRIC_REPRESENTATION_CONTEXT(3)
GLOBAL_UNCERTAINTY_ASSIGNED_CONTEXT((#7614))
GLOBAL_UNIT_ASSIGNED_CONTEXT((#7628,#7630,#7631))
REPRESENTATION_CONTEXT('','3D')
);
#7627=(
GEOMETRIC_REPRESENTATION_CONTEXT(3)
GLOBAL_UNCERTAINTY_ASSIGNED_CONTEXT((#7616))
GLOBAL_UNIT_ASSIGNED_CONTEXT((#7628,#7630,#7631))
REPRESENTATION_CONTEXT('','3D')
);
#7628=(
LENGTH_UNIT()
NAMED_UNIT(*)
SI_UNIT(.MILLI.,.METRE.)
);
#7630=(
NAMED_UNIT(*)
PLANE_ANGLE_UNIT()
SI_UNIT($,.RADIAN.)
);
#7631=(
NAMED_UNIT(*)
SI_UNIT($,.STERADIAN.)
SOLID_ANGLE_UNIT()
);
#7640=SHAPE_DEFINITION_REPRESENTATION(#7650,#7672);
#7650=PRODUCT_DEFINITION_SHAPE('',$,#7683);
#7672=SHAPE_REPRESENTATION('',(#2776),#7625);
#7674=PRODUCT_DEFINITION_CONTEXT('part definition',#7706,'design');
#7683=PRODUCT_DEFINITION('Coil Housing','Coil Housing',#7693,#7674);
#7693=PRODUCT_DEFINITION_FORMATION('',$,#7716);
#7706=APPLICATION_CONTEXT(
'Core Data for Automotive Mechanical Design Process');
#7707=PRODUCT_CONTEXT('part definition',#7706,'mechanical');
#7716=PRODUCT('Coil Housing','Coil Housing',$,(#7707));
#7719=PRESENTATION_STYLE_ASSIGNMENT((#7725));
#7725=SURFACE_STYLE_USAGE(.BOTH.,#7731);
#7731=SURFACE_SIDE_STYLE('',(#7737));
#7737=SURFACE_STYLE_FILL_AREA(#7743);
#7743=FILL_AREA_STYLE('Opaque(20,51,87)',(#7749));
#7749=FILL_AREA_STYLE_COLOUR('Opaque(20,51,87)',#7755);
#7755=COLOUR_RGB('Opaque(20,51,87)',0.0784313725490196,0.2,0.341176470588235);
ENDSEC;
END-ISO-10303-21;
